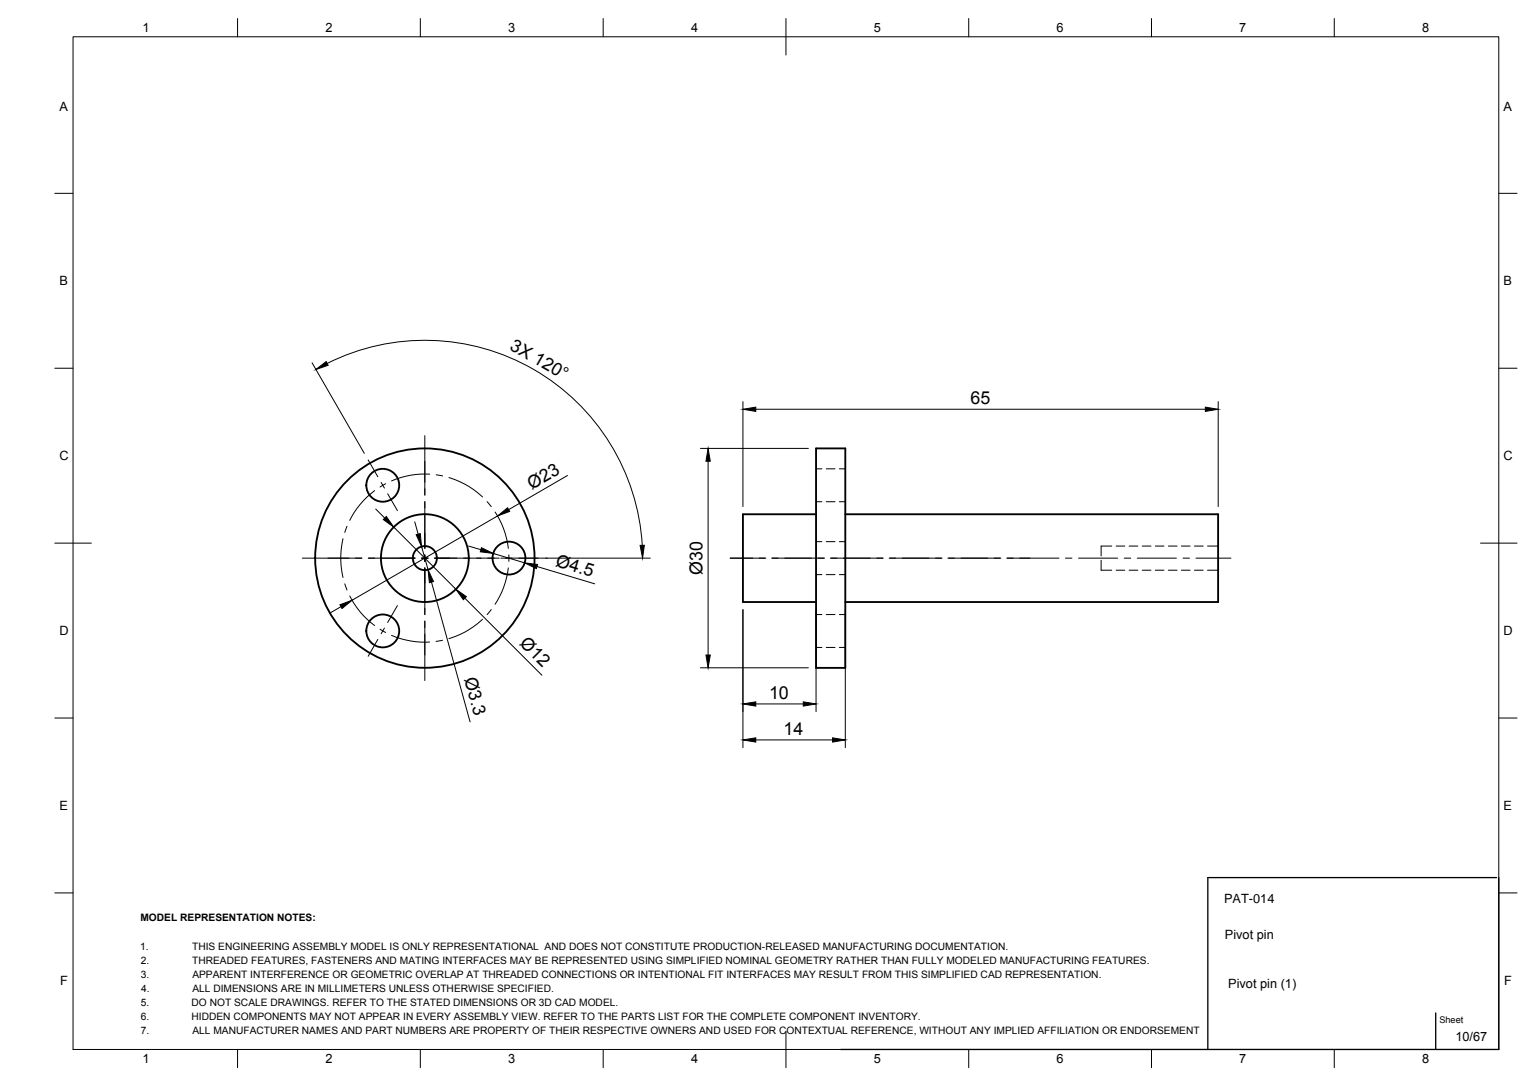
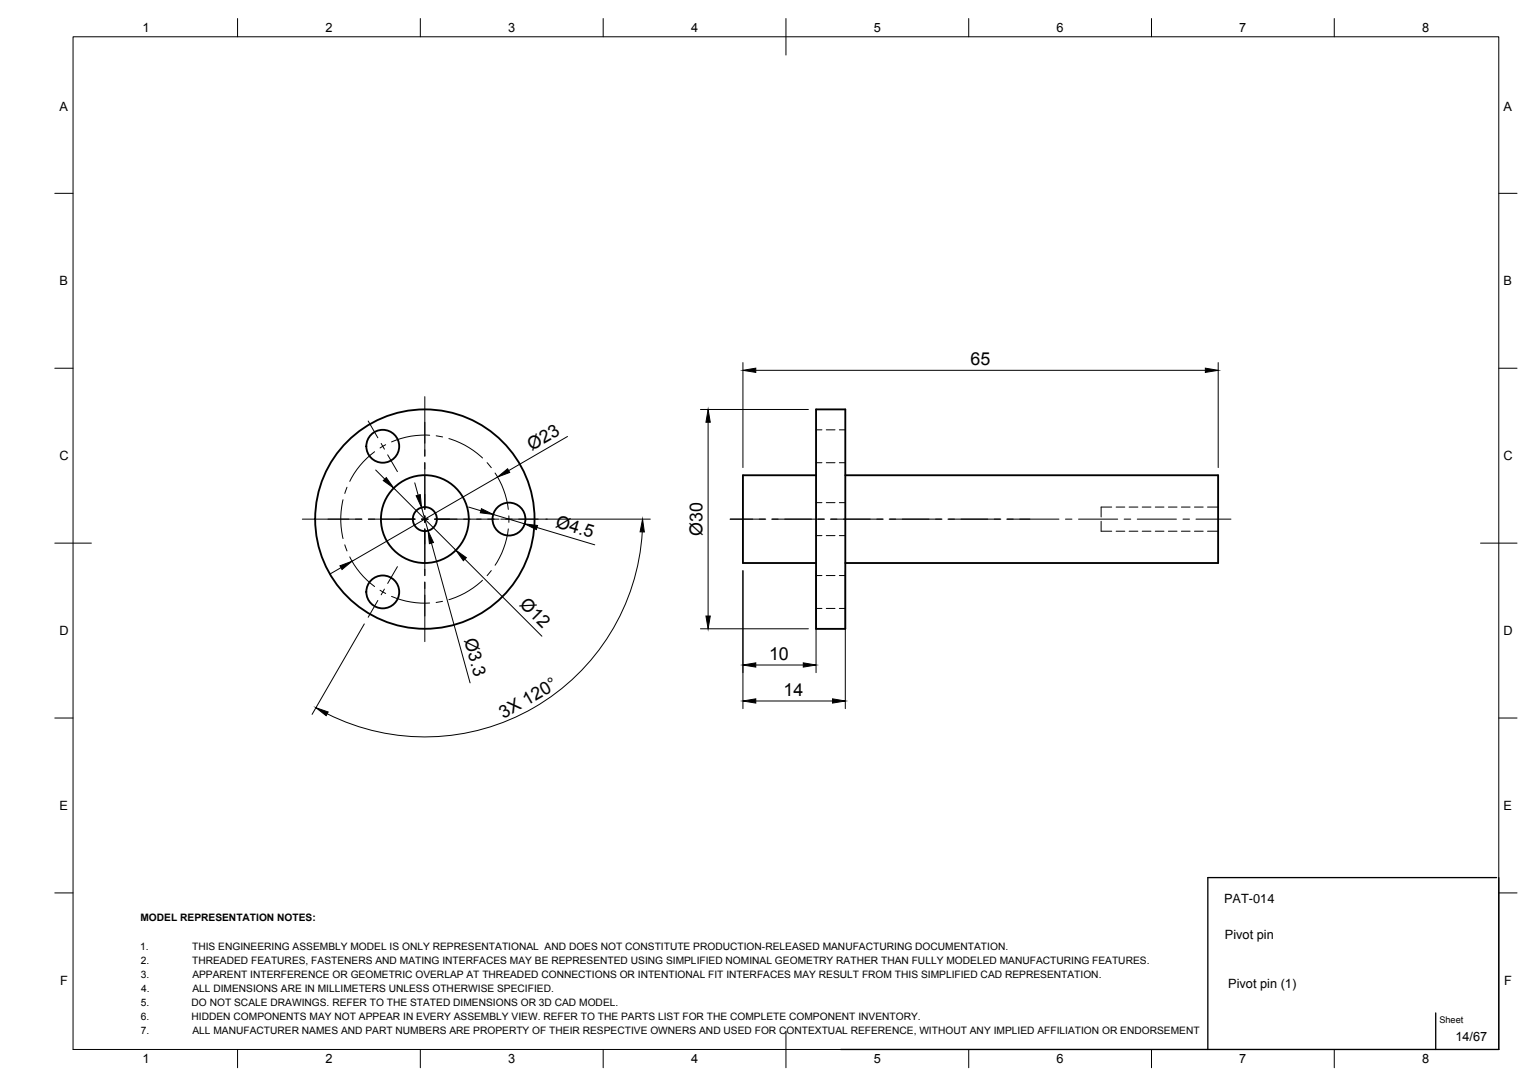
ISO-10303-21;
HEADER;
/* Generated by software containing ST-Developer
 * from STEP Tools, Inc. (www.steptools.com) 
 */

FILE_DESCRIPTION(
/* description */ ('Bin tilter linkage'),
/* implementation_level */ '2;1');

FILE_NAME(
/* name */ 'Pivot pin (1).step',
/* time_stamp */ '2026-10-28T03:26:24-07:00',
/* author */ (''),
/* organization */ (''),
/* preprocessor_version */ 'ST-DEVELOPER v20.2',
/* originating_system */ 'Autodesk Translation Framework v15.17.0.0',
/* authorisation */ '');

FILE_SCHEMA (('AUTOMOTIVE_DESIGN { 1 0 10303 214 3 1 1 }'));
ENDSEC;

DATA;
#10=MECHANICAL_DESIGN_GEOMETRIC_PRESENTATION_REPRESENTATION('',(#871),#23728);
#659=SHAPE_REPRESENTATION_RELATIONSHIP('SRR','None',#24123,#765);
#765=ADVANCED_BREP_SHAPE_REPRESENTATION('',(#985),#23623);
#871=STYLED_ITEM('',(#24765),#985);
#985=MANIFOLD_SOLID_BREP('Body1',#12401);
#1158=FACE_BOUND('',#2834,.T.);
#1159=FACE_BOUND('',#2835,.T.);
#1160=FACE_BOUND('',#2836,.T.);
#1161=FACE_BOUND('',#2837,.T.);
#1162=FACE_BOUND('',#2839,.T.);
#1163=FACE_BOUND('',#2840,.T.);
#1164=FACE_BOUND('',#2841,.T.);
#1165=FACE_BOUND('',#2842,.T.);
#1166=FACE_BOUND('',#2848,.T.);
#1541=PLANE('',#13863);
#1542=PLANE('',#13873);
#1543=PLANE('',#13876);
#1544=PLANE('',#13884);
#1545=PLANE('',#13885);
#1980=FACE_OUTER_BOUND('',#2828,.T.);
#1981=FACE_OUTER_BOUND('',#2829,.T.);
#1982=FACE_OUTER_BOUND('',#2830,.T.);
#1983=FACE_OUTER_BOUND('',#2831,.T.);
#1984=FACE_OUTER_BOUND('',#2832,.T.);
#1985=FACE_OUTER_BOUND('',#2833,.T.);
#1986=FACE_OUTER_BOUND('',#2838,.T.);
#1987=FACE_OUTER_BOUND('',#2843,.T.);
#1988=FACE_OUTER_BOUND('',#2844,.T.);
#1989=FACE_OUTER_BOUND('',#2845,.T.);
#1990=FACE_OUTER_BOUND('',#2846,.T.);
#1991=FACE_OUTER_BOUND('',#2847,.T.);
#2828=EDGE_LOOP('',(#8787,#8788,#8789,#8790));
#2829=EDGE_LOOP('',(#8791));
#2830=EDGE_LOOP('',(#8792,#8793,#8794,#8795));
#2831=EDGE_LOOP('',(#8796,#8797,#8798,#8799));
#2832=EDGE_LOOP('',(#8800,#8801,#8802,#8803));
#2833=EDGE_LOOP('',(#8804));
#2834=EDGE_LOOP('',(#8805));
#2835=EDGE_LOOP('',(#8806));
#2836=EDGE_LOOP('',(#8807));
#2837=EDGE_LOOP('',(#8808));
#2838=EDGE_LOOP('',(#8809));
#2839=EDGE_LOOP('',(#8810));
#2840=EDGE_LOOP('',(#8811));
#2841=EDGE_LOOP('',(#8812));
#2842=EDGE_LOOP('',(#8813));
#2843=EDGE_LOOP('',(#8814,#8815,#8816,#8817));
#2844=EDGE_LOOP('',(#8818,#8819,#8820,#8821));
#2845=EDGE_LOOP('',(#8822,#8823,#8824,#8825));
#2846=EDGE_LOOP('',(#8826));
#2847=EDGE_LOOP('',(#8827));
#2848=EDGE_LOOP('',(#8828));
#3974=LINE('',#20196,#4649);
#3975=LINE('',#20203,#4650);
#3976=LINE('',#20209,#4651);
#3977=LINE('',#20215,#4652);
#3978=LINE('',#20228,#4653);
#3979=LINE('',#20231,#4654);
#3980=LINE('',#20236,#4655);
#4649=VECTOR('',#15971,0.164999999999999);
#4650=VECTOR('',#15980,0.225000000000001);
#4651=VECTOR('',#15987,0.225000000000001);
#4652=VECTOR('',#15994,0.225000000000001);
#4653=VECTOR('',#16011,1.5);
#4654=VECTOR('',#16014,0.600000000000001);
#4655=VECTOR('',#16021,0.600000000000001);
#5281=CIRCLE('',#13861,0.164999999999999);
#5282=CIRCLE('',#13862,0.164999999999999);
#5283=CIRCLE('',#13865,0.225000000000001);
#5284=CIRCLE('',#13866,0.225000000000001);
#5285=CIRCLE('',#13868,0.225000000000001);
#5286=CIRCLE('',#13869,0.225000000000001);
#5287=CIRCLE('',#13871,0.225000000000001);
#5288=CIRCLE('',#13872,0.225000000000001);
#5289=CIRCLE('',#13874,1.5);
#5290=CIRCLE('',#13875,0.600000000000001);
#5291=CIRCLE('',#13877,1.5);
#5292=CIRCLE('',#13878,0.600000000000001);
#5293=CIRCLE('',#13881,0.600000000000001);
#5294=CIRCLE('',#13883,0.600000000000001);
#6095=VERTEX_POINT('',#20193);
#6096=VERTEX_POINT('',#20195);
#6097=VERTEX_POINT('',#20200);
#6098=VERTEX_POINT('',#20202);
#6099=VERTEX_POINT('',#20206);
#6100=VERTEX_POINT('',#20208);
#6101=VERTEX_POINT('',#20212);
#6102=VERTEX_POINT('',#20214);
#6103=VERTEX_POINT('',#20218);
#6104=VERTEX_POINT('',#20220);
#6105=VERTEX_POINT('',#20223);
#6106=VERTEX_POINT('',#20225);
#6107=VERTEX_POINT('',#20230);
#6108=VERTEX_POINT('',#20234);
#7133=EDGE_CURVE('',#6095,#6095,#5281,.T.);
#7134=EDGE_CURVE('',#6095,#6096,#3974,.T.);
#7135=EDGE_CURVE('',#6096,#6096,#5282,.T.);
#7136=EDGE_CURVE('',#6097,#6097,#5283,.T.);
#7137=EDGE_CURVE('',#6097,#6098,#3975,.T.);
#7138=EDGE_CURVE('',#6098,#6098,#5284,.T.);
#7139=EDGE_CURVE('',#6099,#6099,#5285,.T.);
#7140=EDGE_CURVE('',#6099,#6100,#3976,.T.);
#7141=EDGE_CURVE('',#6100,#6100,#5286,.T.);
#7142=EDGE_CURVE('',#6101,#6101,#5287,.T.);
#7143=EDGE_CURVE('',#6101,#6102,#3977,.T.);
#7144=EDGE_CURVE('',#6102,#6102,#5288,.T.);
#7145=EDGE_CURVE('',#6103,#6103,#5289,.T.);
#7146=EDGE_CURVE('',#6104,#6104,#5290,.T.);
#7147=EDGE_CURVE('',#6105,#6105,#5291,.T.);
#7148=EDGE_CURVE('',#6106,#6106,#5292,.T.);
#7149=EDGE_CURVE('',#6103,#6105,#3978,.T.);
#7150=EDGE_CURVE('',#6106,#6107,#3979,.T.);
#7151=EDGE_CURVE('',#6107,#6107,#5293,.T.);
#7152=EDGE_CURVE('',#6108,#6108,#5294,.T.);
#7153=EDGE_CURVE('',#6108,#6104,#3980,.T.);
#8787=ORIENTED_EDGE('',*,*,#7133,.F.);
#8788=ORIENTED_EDGE('',*,*,#7134,.T.);
#8789=ORIENTED_EDGE('',*,*,#7135,.T.);
#8790=ORIENTED_EDGE('',*,*,#7134,.F.);
#8791=ORIENTED_EDGE('',*,*,#7135,.F.);
#8792=ORIENTED_EDGE('',*,*,#7136,.F.);
#8793=ORIENTED_EDGE('',*,*,#7137,.T.);
#8794=ORIENTED_EDGE('',*,*,#7138,.F.);
#8795=ORIENTED_EDGE('',*,*,#7137,.F.);
#8796=ORIENTED_EDGE('',*,*,#7139,.F.);
#8797=ORIENTED_EDGE('',*,*,#7140,.T.);
#8798=ORIENTED_EDGE('',*,*,#7141,.F.);
#8799=ORIENTED_EDGE('',*,*,#7140,.F.);
#8800=ORIENTED_EDGE('',*,*,#7142,.F.);
#8801=ORIENTED_EDGE('',*,*,#7143,.T.);
#8802=ORIENTED_EDGE('',*,*,#7144,.F.);
#8803=ORIENTED_EDGE('',*,*,#7143,.F.);
#8804=ORIENTED_EDGE('',*,*,#7145,.T.);
#8805=ORIENTED_EDGE('',*,*,#7138,.T.);
#8806=ORIENTED_EDGE('',*,*,#7141,.T.);
#8807=ORIENTED_EDGE('',*,*,#7144,.T.);
#8808=ORIENTED_EDGE('',*,*,#7146,.F.);
#8809=ORIENTED_EDGE('',*,*,#7147,.F.);
#8810=ORIENTED_EDGE('',*,*,#7136,.T.);
#8811=ORIENTED_EDGE('',*,*,#7139,.T.);
#8812=ORIENTED_EDGE('',*,*,#7142,.T.);
#8813=ORIENTED_EDGE('',*,*,#7148,.F.);
#8814=ORIENTED_EDGE('',*,*,#7145,.F.);
#8815=ORIENTED_EDGE('',*,*,#7149,.T.);
#8816=ORIENTED_EDGE('',*,*,#7147,.T.);
#8817=ORIENTED_EDGE('',*,*,#7149,.F.);
#8818=ORIENTED_EDGE('',*,*,#7148,.T.);
#8819=ORIENTED_EDGE('',*,*,#7150,.T.);
#8820=ORIENTED_EDGE('',*,*,#7151,.T.);
#8821=ORIENTED_EDGE('',*,*,#7150,.F.);
#8822=ORIENTED_EDGE('',*,*,#7152,.F.);
#8823=ORIENTED_EDGE('',*,*,#7153,.T.);
#8824=ORIENTED_EDGE('',*,*,#7146,.T.);
#8825=ORIENTED_EDGE('',*,*,#7153,.F.);
#8826=ORIENTED_EDGE('',*,*,#7152,.T.);
#8827=ORIENTED_EDGE('',*,*,#7151,.F.);
#8828=ORIENTED_EDGE('',*,*,#7133,.T.);
#11308=CYLINDRICAL_SURFACE('',#13860,0.164999999999999);
#11309=CYLINDRICAL_SURFACE('',#13864,0.225000000000001);
#11310=CYLINDRICAL_SURFACE('',#13867,0.225000000000001);
#11311=CYLINDRICAL_SURFACE('',#13870,0.225000000000001);
#11312=CYLINDRICAL_SURFACE('',#13879,1.5);
#11313=CYLINDRICAL_SURFACE('',#13880,0.600000000000001);
#11314=CYLINDRICAL_SURFACE('',#13882,0.600000000000001);
#11705=ADVANCED_FACE('',(#1980),#11308,.F.);
#11706=ADVANCED_FACE('',(#1981),#1541,.F.);
#11707=ADVANCED_FACE('',(#1982),#11309,.F.);
#11708=ADVANCED_FACE('',(#1983),#11310,.F.);
#11709=ADVANCED_FACE('',(#1984),#11311,.F.);
#11710=ADVANCED_FACE('',(#1985,#1158,#1159,#1160,#1161),#1542,.T.);
#11711=ADVANCED_FACE('',(#1986,#1162,#1163,#1164,#1165),#1543,.F.);
#11712=ADVANCED_FACE('',(#1987),#11312,.T.);
#11713=ADVANCED_FACE('',(#1988),#11313,.T.);
#11714=ADVANCED_FACE('',(#1989),#11314,.T.);
#11715=ADVANCED_FACE('',(#1990),#1544,.T.);
#11716=ADVANCED_FACE('',(#1991,#1166),#1545,.F.);
#12401=CLOSED_SHELL('',(#11705,#11706,#11707,#11708,#11709,#11710,#11711,
#11712,#11713,#11714,#11715,#11716));
#13859=AXIS2_PLACEMENT_3D('',#20191,#15965,#15966);
#13860=AXIS2_PLACEMENT_3D('',#20192,#15967,#15968);
#13861=AXIS2_PLACEMENT_3D('',#20194,#15969,#15970);
#13862=AXIS2_PLACEMENT_3D('',#20197,#15972,#15973);
#13863=AXIS2_PLACEMENT_3D('',#20198,#15974,#15975);
#13864=AXIS2_PLACEMENT_3D('',#20199,#15976,#15977);
#13865=AXIS2_PLACEMENT_3D('',#20201,#15978,#15979);
#13866=AXIS2_PLACEMENT_3D('',#20204,#15981,#15982);
#13867=AXIS2_PLACEMENT_3D('',#20205,#15983,#15984);
#13868=AXIS2_PLACEMENT_3D('',#20207,#15985,#15986);
#13869=AXIS2_PLACEMENT_3D('',#20210,#15988,#15989);
#13870=AXIS2_PLACEMENT_3D('',#20211,#15990,#15991);
#13871=AXIS2_PLACEMENT_3D('',#20213,#15992,#15993);
#13872=AXIS2_PLACEMENT_3D('',#20216,#15995,#15996);
#13873=AXIS2_PLACEMENT_3D('',#20217,#15997,#15998);
#13874=AXIS2_PLACEMENT_3D('',#20219,#15999,#16000);
#13875=AXIS2_PLACEMENT_3D('',#20221,#16001,#16002);
#13876=AXIS2_PLACEMENT_3D('',#20222,#16003,#16004);
#13877=AXIS2_PLACEMENT_3D('',#20224,#16005,#16006);
#13878=AXIS2_PLACEMENT_3D('',#20226,#16007,#16008);
#13879=AXIS2_PLACEMENT_3D('',#20227,#16009,#16010);
#13880=AXIS2_PLACEMENT_3D('',#20229,#16012,#16013);
#13881=AXIS2_PLACEMENT_3D('',#20232,#16015,#16016);
#13882=AXIS2_PLACEMENT_3D('',#20233,#16017,#16018);
#13883=AXIS2_PLACEMENT_3D('',#20235,#16019,#16020);
#13884=AXIS2_PLACEMENT_3D('',#20237,#16022,#16023);
#13885=AXIS2_PLACEMENT_3D('',#20238,#16024,#16025);
#15965=DIRECTION('axis',(0.,0.,1.));
#15966=DIRECTION('refdir',(1.,0.,0.));
#15967=DIRECTION('center_axis',(0.,1.,0.));
#15968=DIRECTION('ref_axis',(1.,0.,0.));
#15969=DIRECTION('center_axis',(0.,1.,0.));
#15970=DIRECTION('ref_axis',(1.,0.,0.));
#15971=DIRECTION('',(0.,1.,0.));
#15972=DIRECTION('center_axis',(0.,1.,0.));
#15973=DIRECTION('ref_axis',(1.,0.,0.));
#15974=DIRECTION('center_axis',(0.,1.,0.));
#15975=DIRECTION('ref_axis',(1.,0.,0.));
#15976=DIRECTION('center_axis',(0.,1.,0.));
#15977=DIRECTION('ref_axis',(1.,0.,0.));
#15978=DIRECTION('center_axis',(0.,1.,0.));
#15979=DIRECTION('ref_axis',(1.,0.,0.));
#15980=DIRECTION('',(0.,1.,0.));
#15981=DIRECTION('center_axis',(0.,-1.,0.));
#15982=DIRECTION('ref_axis',(1.,0.,0.));
#15983=DIRECTION('center_axis',(0.,1.,0.));
#15984=DIRECTION('ref_axis',(1.,0.,0.));
#15985=DIRECTION('center_axis',(0.,1.,0.));
#15986=DIRECTION('ref_axis',(1.,0.,0.));
#15987=DIRECTION('',(0.,1.,0.));
#15988=DIRECTION('center_axis',(0.,-1.,0.));
#15989=DIRECTION('ref_axis',(1.,0.,0.));
#15990=DIRECTION('center_axis',(0.,1.,0.));
#15991=DIRECTION('ref_axis',(1.,0.,0.));
#15992=DIRECTION('center_axis',(0.,1.,0.));
#15993=DIRECTION('ref_axis',(1.,0.,0.));
#15994=DIRECTION('',(0.,1.,0.));
#15995=DIRECTION('center_axis',(0.,-1.,0.));
#15996=DIRECTION('ref_axis',(1.,0.,0.));
#15997=DIRECTION('center_axis',(0.,1.,0.));
#15998=DIRECTION('ref_axis',(1.,0.,0.));
#15999=DIRECTION('center_axis',(0.,1.,0.));
#16000=DIRECTION('ref_axis',(1.,0.,0.));
#16001=DIRECTION('center_axis',(0.,1.,0.));
#16002=DIRECTION('ref_axis',(1.,0.,0.));
#16003=DIRECTION('center_axis',(0.,1.,0.));
#16004=DIRECTION('ref_axis',(1.,0.,0.));
#16005=DIRECTION('center_axis',(0.,1.,0.));
#16006=DIRECTION('ref_axis',(1.,0.,0.));
#16007=DIRECTION('center_axis',(0.,-1.,0.));
#16008=DIRECTION('ref_axis',(1.,0.,0.));
#16009=DIRECTION('center_axis',(0.,1.,0.));
#16010=DIRECTION('ref_axis',(1.,0.,0.));
#16011=DIRECTION('',(0.,-1.,0.));
#16012=DIRECTION('center_axis',(0.,1.,0.));
#16013=DIRECTION('ref_axis',(1.,0.,0.));
#16014=DIRECTION('',(0.,-1.,0.));
#16015=DIRECTION('center_axis',(0.,1.,0.));
#16016=DIRECTION('ref_axis',(1.,0.,0.));
#16017=DIRECTION('center_axis',(0.,1.,0.));
#16018=DIRECTION('ref_axis',(1.,0.,0.));
#16019=DIRECTION('center_axis',(0.,1.,0.));
#16020=DIRECTION('ref_axis',(1.,0.,0.));
#16021=DIRECTION('',(0.,-1.,0.));
#16022=DIRECTION('center_axis',(0.,1.,0.));
#16023=DIRECTION('ref_axis',(1.,0.,0.));
#16024=DIRECTION('center_axis',(0.,1.,0.));
#16025=DIRECTION('ref_axis',(1.,0.,0.));
#20191=CARTESIAN_POINT('',(0.,0.,0.));
#20192=CARTESIAN_POINT('Origin',(18.,-1.1,15.));
#20193=CARTESIAN_POINT('',(17.835,-1.,15.));
#20194=CARTESIAN_POINT('Origin',(18.,-1.,15.));
#20195=CARTESIAN_POINT('',(17.835,0.6,15.));
#20196=CARTESIAN_POINT('',(17.835,-1.1,15.));
#20197=CARTESIAN_POINT('Origin',(18.,0.6,15.));
#20198=CARTESIAN_POINT('Origin',(18.,0.6,15.));
#20199=CARTESIAN_POINT('Origin',(19.15,4.,15.));
#20200=CARTESIAN_POINT('',(18.925,4.1,15.));
#20201=CARTESIAN_POINT('Origin',(19.15,4.1,15.));
#20202=CARTESIAN_POINT('',(18.925,4.5,15.));
#20203=CARTESIAN_POINT('',(18.925,4.,15.));
#20204=CARTESIAN_POINT('Origin',(19.15,4.5,15.));
#20205=CARTESIAN_POINT('Origin',(17.425,4.,15.9959292143521));
#20206=CARTESIAN_POINT('',(17.2,4.1,15.9959292143521));
#20207=CARTESIAN_POINT('Origin',(17.425,4.1,15.9959292143521));
#20208=CARTESIAN_POINT('',(17.2,4.5,15.9959292143521));
#20209=CARTESIAN_POINT('',(17.2,4.,15.9959292143521));
#20210=CARTESIAN_POINT('Origin',(17.425,4.5,15.9959292143521));
#20211=CARTESIAN_POINT('Origin',(17.425,4.,14.0040707856479));
#20212=CARTESIAN_POINT('',(17.2,4.1,14.0040707856479));
#20213=CARTESIAN_POINT('Origin',(17.425,4.1,14.0040707856479));
#20214=CARTESIAN_POINT('',(17.2,4.5,14.0040707856479));
#20215=CARTESIAN_POINT('',(17.2,4.,14.0040707856479));
#20216=CARTESIAN_POINT('Origin',(17.425,4.5,14.0040707856479));
#20217=CARTESIAN_POINT('Origin',(18.,4.5,15.));
#20218=CARTESIAN_POINT('',(16.5,4.5,15.));
#20219=CARTESIAN_POINT('Origin',(18.,4.5,15.));
#20220=CARTESIAN_POINT('',(17.4,4.5,15.));
#20221=CARTESIAN_POINT('Origin',(18.,4.5,15.));
#20222=CARTESIAN_POINT('Origin',(18.,4.1,15.));
#20223=CARTESIAN_POINT('',(16.5,4.1,15.));
#20224=CARTESIAN_POINT('Origin',(18.,4.1,15.));
#20225=CARTESIAN_POINT('',(17.4,4.1,15.));
#20226=CARTESIAN_POINT('Origin',(18.,4.1,15.));
#20227=CARTESIAN_POINT('Origin',(18.,4.1,15.));
#20228=CARTESIAN_POINT('',(16.5,4.1,15.));
#20229=CARTESIAN_POINT('Origin',(18.,-1.,15.));
#20230=CARTESIAN_POINT('',(17.4,-1.,15.));
#20231=CARTESIAN_POINT('',(17.4,-1.,15.));
#20232=CARTESIAN_POINT('Origin',(18.,-1.,15.));
#20233=CARTESIAN_POINT('Origin',(18.,-1.,15.));
#20234=CARTESIAN_POINT('',(17.4,5.5,15.));
#20235=CARTESIAN_POINT('Origin',(18.,5.5,15.));
#20236=CARTESIAN_POINT('',(17.4,-1.,15.));
#20237=CARTESIAN_POINT('Origin',(18.,5.5,15.));
#20238=CARTESIAN_POINT('Origin',(18.,-1.,15.));
#23506=UNCERTAINTY_MEASURE_WITH_UNIT(LENGTH_MEASURE(0.001),#23729,
'DISTANCE_ACCURACY_VALUE',
'Maximum model space distance between geometric entities at asserted c
onnectivities');
#23611=UNCERTAINTY_MEASURE_WITH_UNIT(LENGTH_MEASURE(0.001),#23729,
'DISTANCE_ACCURACY_VALUE',
'Maximum model space distance between geometric entities at asserted c
onnectivities');
#23623=(
GEOMETRIC_REPRESENTATION_CONTEXT(3)
GLOBAL_UNCERTAINTY_ASSIGNED_CONTEXT((#23506))
GLOBAL_UNIT_ASSIGNED_CONTEXT((#23729,#23731,#23732))
REPRESENTATION_CONTEXT('','3D')
);
#23728=(
GEOMETRIC_REPRESENTATION_CONTEXT(3)
GLOBAL_UNCERTAINTY_ASSIGNED_CONTEXT((#23611))
GLOBAL_UNIT_ASSIGNED_CONTEXT((#23729,#23731,#23732))
REPRESENTATION_CONTEXT('','3D')
);
#23729=(
LENGTH_UNIT()
NAMED_UNIT(*)
SI_UNIT(.CENTI.,.METRE.)
);
#23731=(
NAMED_UNIT(*)
PLANE_ANGLE_UNIT()
SI_UNIT($,.RADIAN.)
);
#23732=(
NAMED_UNIT(*)
SI_UNIT($,.STERADIAN.)
SOLID_ANGLE_UNIT()
);
#23744=SHAPE_DEFINITION_REPRESENTATION(#23860,#24123);
#23860=PRODUCT_DEFINITION_SHAPE('',$,#24240);
#24123=SHAPE_REPRESENTATION('',(#13859),#23623);
#24228=PRODUCT_DEFINITION_CONTEXT('part definition',#24578,'design');
#24240=PRODUCT_DEFINITION('Pivot pin (1)','Pivot pin (1)',#24356,#24228);
#24356=PRODUCT_DEFINITION_FORMATION('',$,#24591);
#24578=APPLICATION_CONTEXT(
'Core Data for Automotive Mechanical Design Process');
#24579=PRODUCT_CONTEXT('part definition',#24578,'mechanical');
#24591=PRODUCT('Pivot pin (1)','Pivot pin (1)','Pivot pin (1)',(#24579));
#24759=COLOUR_RGB('Grey',0.48,0.52,0.57);
#24760=FILL_AREA_STYLE_COLOUR('',#24759);
#24761=FILL_AREA_STYLE('',(#24760));
#24762=SURFACE_STYLE_FILL_AREA(#24761);
#24763=SURFACE_SIDE_STYLE('',(#24762));
#24764=SURFACE_STYLE_USAGE(.BOTH.,#24763);
#24765=PRESENTATION_STYLE_ASSIGNMENT((#24764));
ENDSEC;
END-ISO-10303-21;
